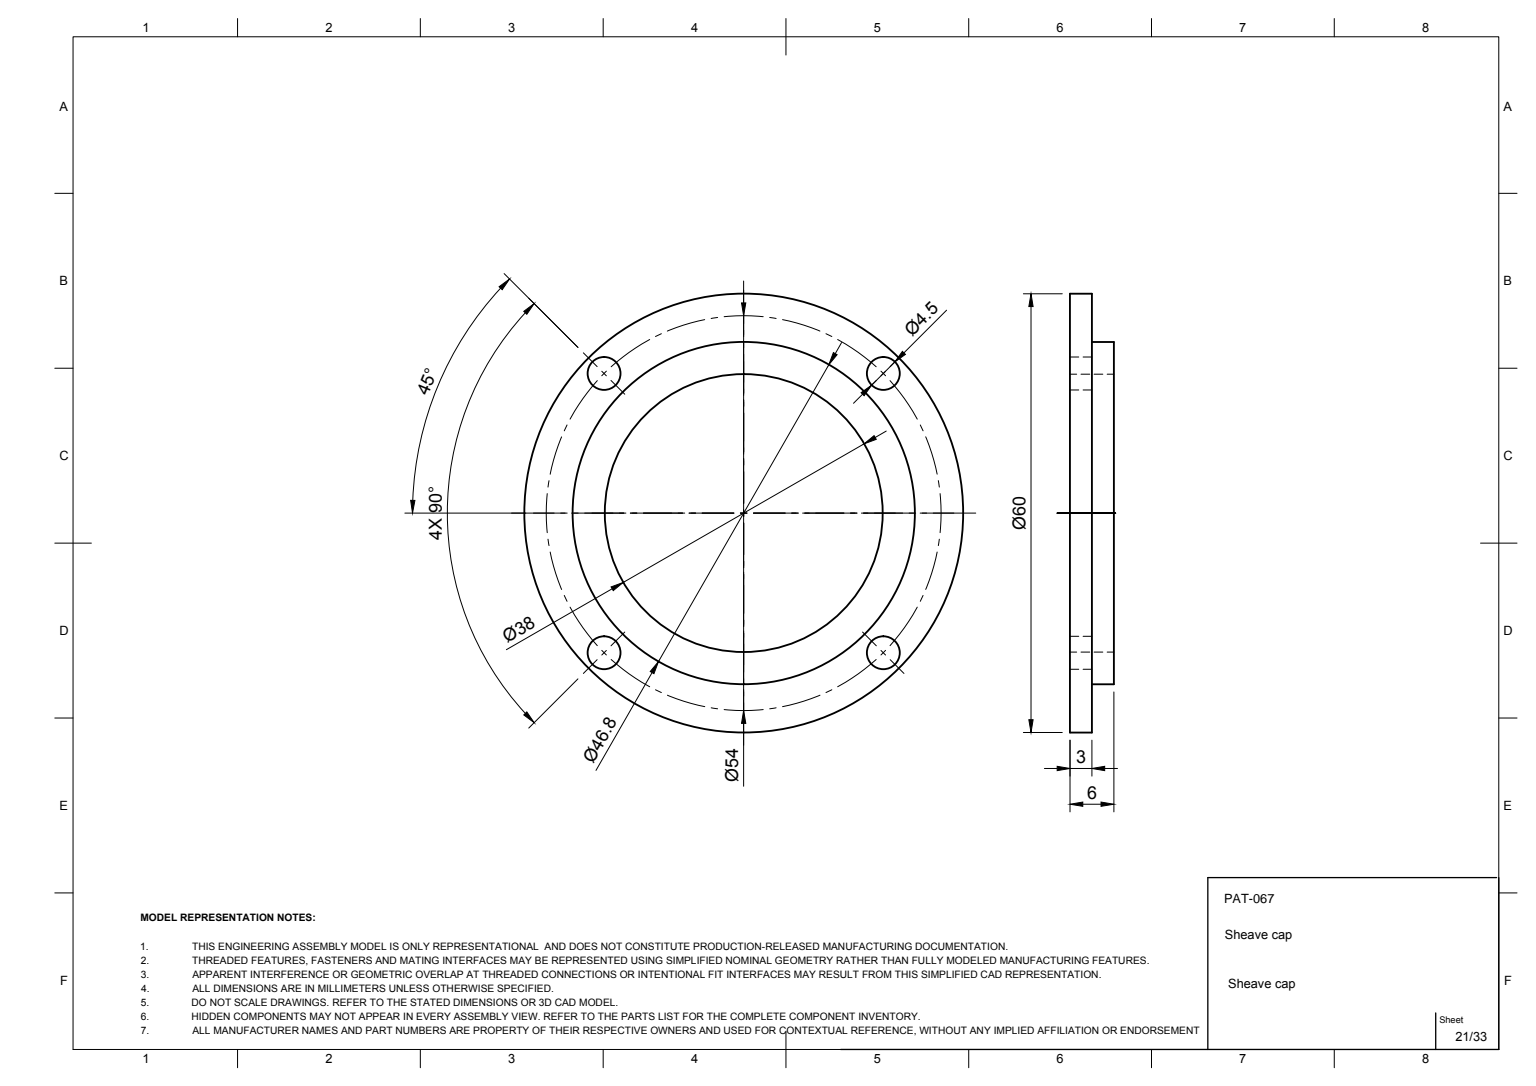
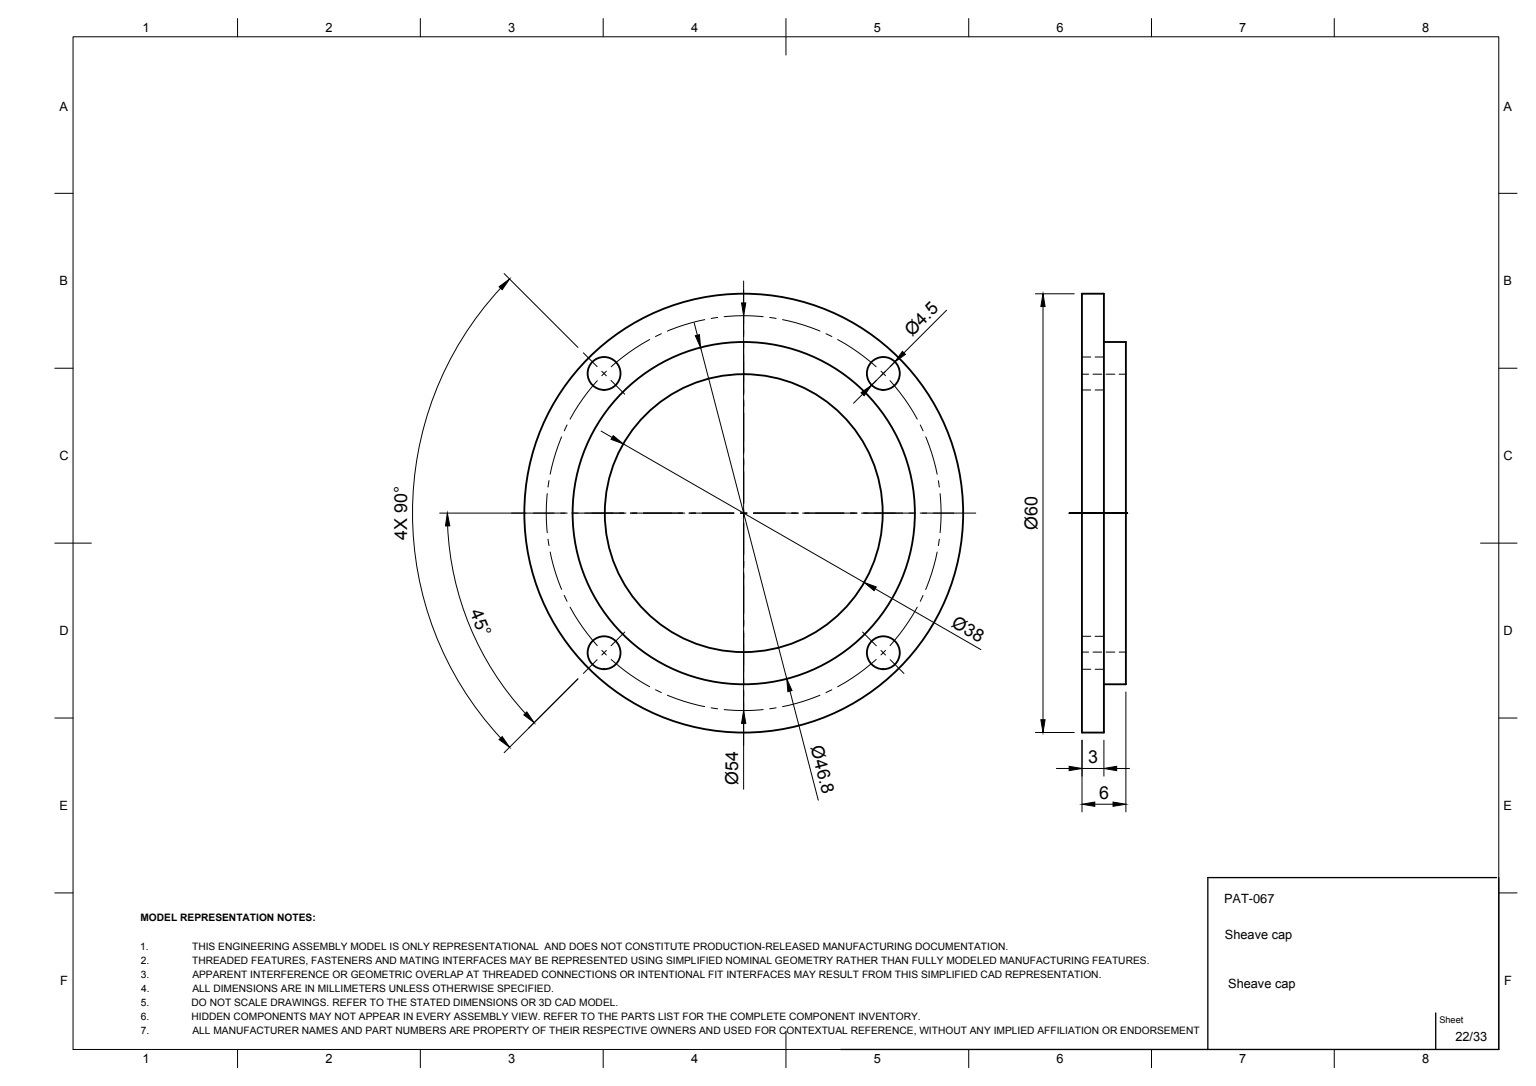
ISO-10303-21;
HEADER;
/* Generated by software containing ST-Developer
 * from STEP Tools, Inc. (www.steptools.com) 
 */

FILE_DESCRIPTION(
/* description */ ('Lifting hook block with sheave'),
/* implementation_level */ '2;1');

FILE_NAME(
/* name */ 'Sheave cap.step',
/* time_stamp */ '2026-10-28T03:23:54-07:00',
/* author */ (''),
/* organization */ (''),
/* preprocessor_version */ 'ST-DEVELOPER v20.2',
/* originating_system */ 'Autodesk Translation Framework v15.17.0.0',
/* authorisation */ '');

FILE_SCHEMA (('AUTOMOTIVE_DESIGN { 1 0 10303 214 3 1 1 }'));
ENDSEC;

DATA;
#10=MECHANICAL_DESIGN_GEOMETRIC_PRESENTATION_REPRESENTATION('',(#369),#9391);
#309=SHAPE_REPRESENTATION_RELATIONSHIP('SRR','None',#9541,#339);
#339=ADVANCED_BREP_SHAPE_REPRESENTATION('',(#405),#9376);
#369=STYLED_ITEM('',(#9773),#405);
#405=MANIFOLD_SOLID_BREP('Body1',#4907);
#612=LINE('',#8395,#900);
#613=LINE('',#8401,#901);
#614=LINE('',#8407,#902);
#615=LINE('',#8413,#903);
#616=LINE('',#8419,#904);
#617=LINE('',#8426,#905);
#618=LINE('',#8432,#906);
#900=VECTOR('',#6869,0.225);
#901=VECTOR('',#6876,0.225);
#902=VECTOR('',#6883,0.225);
#903=VECTOR('',#6890,0.225);
#904=VECTOR('',#6897,2.34);
#905=VECTOR('',#6906,1.9);
#906=VECTOR('',#6913,3.);
#1067=CYLINDRICAL_SURFACE('',#5633,0.225);
#1068=CYLINDRICAL_SURFACE('',#5636,0.225);
#1069=CYLINDRICAL_SURFACE('',#5639,0.225);
#1070=CYLINDRICAL_SURFACE('',#5642,0.225);
#1071=CYLINDRICAL_SURFACE('',#5645,2.34);
#1072=CYLINDRICAL_SURFACE('',#5650,1.9);
#1073=CYLINDRICAL_SURFACE('',#5652,3.);
#1180=FACE_BOUND('',#1757,.T.);
#1181=FACE_BOUND('',#1761,.T.);
#1182=FACE_BOUND('',#1762,.T.);
#1183=FACE_BOUND('',#1763,.T.);
#1184=FACE_BOUND('',#1764,.T.);
#1185=FACE_BOUND('',#1765,.T.);
#1186=FACE_BOUND('',#1767,.T.);
#1187=FACE_BOUND('',#1768,.T.);
#1188=FACE_BOUND('',#1769,.T.);
#1189=FACE_BOUND('',#1770,.T.);
#1190=FACE_BOUND('',#1771,.T.);
#1389=FACE_OUTER_BOUND('',#1751,.T.);
#1390=FACE_OUTER_BOUND('',#1752,.T.);
#1391=FACE_OUTER_BOUND('',#1753,.T.);
#1392=FACE_OUTER_BOUND('',#1754,.T.);
#1393=FACE_OUTER_BOUND('',#1755,.T.);
#1394=FACE_OUTER_BOUND('',#1756,.T.);
#1395=FACE_OUTER_BOUND('',#1758,.T.);
#1396=FACE_OUTER_BOUND('',#1759,.T.);
#1397=FACE_OUTER_BOUND('',#1760,.T.);
#1398=FACE_OUTER_BOUND('',#1766,.T.);
#1751=EDGE_LOOP('',(#3950,#3951,#3952,#3953));
#1752=EDGE_LOOP('',(#3954,#3955,#3956,#3957));
#1753=EDGE_LOOP('',(#3958,#3959,#3960,#3961));
#1754=EDGE_LOOP('',(#3962,#3963,#3964,#3965));
#1755=EDGE_LOOP('',(#3966,#3967,#3968,#3969));
#1756=EDGE_LOOP('',(#3970));
#1757=EDGE_LOOP('',(#3971));
#1758=EDGE_LOOP('',(#3972,#3973,#3974,#3975));
#1759=EDGE_LOOP('',(#3976,#3977,#3978,#3979));
#1760=EDGE_LOOP('',(#3980));
#1761=EDGE_LOOP('',(#3981));
#1762=EDGE_LOOP('',(#3982));
#1763=EDGE_LOOP('',(#3983));
#1764=EDGE_LOOP('',(#3984));
#1765=EDGE_LOOP('',(#3985));
#1766=EDGE_LOOP('',(#3986));
#1767=EDGE_LOOP('',(#3987));
#1768=EDGE_LOOP('',(#3988));
#1769=EDGE_LOOP('',(#3989));
#1770=EDGE_LOOP('',(#3990));
#1771=EDGE_LOOP('',(#3991));
#2075=CIRCLE('',#5634,0.225);
#2076=CIRCLE('',#5635,0.225);
#2077=CIRCLE('',#5637,0.225);
#2078=CIRCLE('',#5638,0.225);
#2079=CIRCLE('',#5640,0.225);
#2080=CIRCLE('',#5641,0.225);
#2081=CIRCLE('',#5643,0.225);
#2082=CIRCLE('',#5644,0.225);
#2083=CIRCLE('',#5646,2.34);
#2084=CIRCLE('',#5647,2.34);
#2085=CIRCLE('',#5649,1.9);
#2086=CIRCLE('',#5651,1.9);
#2087=CIRCLE('',#5653,3.);
#2088=CIRCLE('',#5654,3.);
#2444=VERTEX_POINT('',#8392);
#2445=VERTEX_POINT('',#8394);
#2446=VERTEX_POINT('',#8398);
#2447=VERTEX_POINT('',#8400);
#2448=VERTEX_POINT('',#8404);
#2449=VERTEX_POINT('',#8406);
#2450=VERTEX_POINT('',#8410);
#2451=VERTEX_POINT('',#8412);
#2452=VERTEX_POINT('',#8416);
#2453=VERTEX_POINT('',#8418);
#2454=VERTEX_POINT('',#8422);
#2455=VERTEX_POINT('',#8425);
#2456=VERTEX_POINT('',#8429);
#2457=VERTEX_POINT('',#8431);
#2979=EDGE_CURVE('',#2444,#2444,#2075,.T.);
#2980=EDGE_CURVE('',#2444,#2445,#612,.T.);
#2981=EDGE_CURVE('',#2445,#2445,#2076,.T.);
#2982=EDGE_CURVE('',#2446,#2446,#2077,.T.);
#2983=EDGE_CURVE('',#2446,#2447,#613,.T.);
#2984=EDGE_CURVE('',#2447,#2447,#2078,.T.);
#2985=EDGE_CURVE('',#2448,#2448,#2079,.T.);
#2986=EDGE_CURVE('',#2448,#2449,#614,.T.);
#2987=EDGE_CURVE('',#2449,#2449,#2080,.T.);
#2988=EDGE_CURVE('',#2450,#2450,#2081,.T.);
#2989=EDGE_CURVE('',#2450,#2451,#615,.T.);
#2990=EDGE_CURVE('',#2451,#2451,#2082,.T.);
#2991=EDGE_CURVE('',#2452,#2452,#2083,.T.);
#2992=EDGE_CURVE('',#2452,#2453,#616,.T.);
#2993=EDGE_CURVE('',#2453,#2453,#2084,.T.);
#2994=EDGE_CURVE('',#2454,#2454,#2085,.T.);
#2995=EDGE_CURVE('',#2454,#2455,#617,.T.);
#2996=EDGE_CURVE('',#2455,#2455,#2086,.T.);
#2997=EDGE_CURVE('',#2456,#2456,#2087,.T.);
#2998=EDGE_CURVE('',#2456,#2457,#618,.T.);
#2999=EDGE_CURVE('',#2457,#2457,#2088,.T.);
#3950=ORIENTED_EDGE('',*,*,#2979,.F.);
#3951=ORIENTED_EDGE('',*,*,#2980,.T.);
#3952=ORIENTED_EDGE('',*,*,#2981,.F.);
#3953=ORIENTED_EDGE('',*,*,#2980,.F.);
#3954=ORIENTED_EDGE('',*,*,#2982,.F.);
#3955=ORIENTED_EDGE('',*,*,#2983,.T.);
#3956=ORIENTED_EDGE('',*,*,#2984,.F.);
#3957=ORIENTED_EDGE('',*,*,#2983,.F.);
#3958=ORIENTED_EDGE('',*,*,#2985,.F.);
#3959=ORIENTED_EDGE('',*,*,#2986,.T.);
#3960=ORIENTED_EDGE('',*,*,#2987,.F.);
#3961=ORIENTED_EDGE('',*,*,#2986,.F.);
#3962=ORIENTED_EDGE('',*,*,#2988,.F.);
#3963=ORIENTED_EDGE('',*,*,#2989,.T.);
#3964=ORIENTED_EDGE('',*,*,#2990,.F.);
#3965=ORIENTED_EDGE('',*,*,#2989,.F.);
#3966=ORIENTED_EDGE('',*,*,#2991,.F.);
#3967=ORIENTED_EDGE('',*,*,#2992,.T.);
#3968=ORIENTED_EDGE('',*,*,#2993,.F.);
#3969=ORIENTED_EDGE('',*,*,#2992,.F.);
#3970=ORIENTED_EDGE('',*,*,#2991,.T.);
#3971=ORIENTED_EDGE('',*,*,#2994,.T.);
#3972=ORIENTED_EDGE('',*,*,#2994,.F.);
#3973=ORIENTED_EDGE('',*,*,#2995,.T.);
#3974=ORIENTED_EDGE('',*,*,#2996,.T.);
#3975=ORIENTED_EDGE('',*,*,#2995,.F.);
#3976=ORIENTED_EDGE('',*,*,#2997,.F.);
#3977=ORIENTED_EDGE('',*,*,#2998,.T.);
#3978=ORIENTED_EDGE('',*,*,#2999,.T.);
#3979=ORIENTED_EDGE('',*,*,#2998,.F.);
#3980=ORIENTED_EDGE('',*,*,#2997,.T.);
#3981=ORIENTED_EDGE('',*,*,#2993,.T.);
#3982=ORIENTED_EDGE('',*,*,#2990,.T.);
#3983=ORIENTED_EDGE('',*,*,#2987,.T.);
#3984=ORIENTED_EDGE('',*,*,#2984,.T.);
#3985=ORIENTED_EDGE('',*,*,#2981,.T.);
#3986=ORIENTED_EDGE('',*,*,#2999,.F.);
#3987=ORIENTED_EDGE('',*,*,#2996,.F.);
#3988=ORIENTED_EDGE('',*,*,#2988,.T.);
#3989=ORIENTED_EDGE('',*,*,#2985,.T.);
#3990=ORIENTED_EDGE('',*,*,#2982,.T.);
#3991=ORIENTED_EDGE('',*,*,#2979,.T.);
#4541=PLANE('',#5648);
#4542=PLANE('',#5655);
#4543=PLANE('',#5656);
#4765=ADVANCED_FACE('',(#1389),#1067,.F.);
#4766=ADVANCED_FACE('',(#1390),#1068,.F.);
#4767=ADVANCED_FACE('',(#1391),#1069,.F.);
#4768=ADVANCED_FACE('',(#1392),#1070,.F.);
#4769=ADVANCED_FACE('',(#1393),#1071,.T.);
#4770=ADVANCED_FACE('',(#1394,#1180),#4541,.T.);
#4771=ADVANCED_FACE('',(#1395),#1072,.F.);
#4772=ADVANCED_FACE('',(#1396),#1073,.T.);
#4773=ADVANCED_FACE('',(#1397,#1181,#1182,#1183,#1184,#1185),#4542,.T.);
#4774=ADVANCED_FACE('',(#1398,#1186,#1187,#1188,#1189,#1190),#4543,.F.);
#4907=CLOSED_SHELL('',(#4765,#4766,#4767,#4768,#4769,#4770,#4771,#4772,
#4773,#4774));
#5632=AXIS2_PLACEMENT_3D('',#8390,#6863,#6864);
#5633=AXIS2_PLACEMENT_3D('',#8391,#6865,#6866);
#5634=AXIS2_PLACEMENT_3D('',#8393,#6867,#6868);
#5635=AXIS2_PLACEMENT_3D('',#8396,#6870,#6871);
#5636=AXIS2_PLACEMENT_3D('',#8397,#6872,#6873);
#5637=AXIS2_PLACEMENT_3D('',#8399,#6874,#6875);
#5638=AXIS2_PLACEMENT_3D('',#8402,#6877,#6878);
#5639=AXIS2_PLACEMENT_3D('',#8403,#6879,#6880);
#5640=AXIS2_PLACEMENT_3D('',#8405,#6881,#6882);
#5641=AXIS2_PLACEMENT_3D('',#8408,#6884,#6885);
#5642=AXIS2_PLACEMENT_3D('',#8409,#6886,#6887);
#5643=AXIS2_PLACEMENT_3D('',#8411,#6888,#6889);
#5644=AXIS2_PLACEMENT_3D('',#8414,#6891,#6892);
#5645=AXIS2_PLACEMENT_3D('',#8415,#6893,#6894);
#5646=AXIS2_PLACEMENT_3D('',#8417,#6895,#6896);
#5647=AXIS2_PLACEMENT_3D('',#8420,#6898,#6899);
#5648=AXIS2_PLACEMENT_3D('',#8421,#6900,#6901);
#5649=AXIS2_PLACEMENT_3D('',#8423,#6902,#6903);
#5650=AXIS2_PLACEMENT_3D('',#8424,#6904,#6905);
#5651=AXIS2_PLACEMENT_3D('',#8427,#6907,#6908);
#5652=AXIS2_PLACEMENT_3D('',#8428,#6909,#6910);
#5653=AXIS2_PLACEMENT_3D('',#8430,#6911,#6912);
#5654=AXIS2_PLACEMENT_3D('',#8433,#6914,#6915);
#5655=AXIS2_PLACEMENT_3D('',#8434,#6916,#6917);
#5656=AXIS2_PLACEMENT_3D('',#8435,#6918,#6919);
#6863=DIRECTION('axis',(0.,0.,1.));
#6864=DIRECTION('refdir',(1.,0.,0.));
#6865=DIRECTION('center_axis',(0.,1.,0.));
#6866=DIRECTION('ref_axis',(1.,0.,0.));
#6867=DIRECTION('center_axis',(0.,1.,0.));
#6868=DIRECTION('ref_axis',(1.,0.,0.));
#6869=DIRECTION('',(0.,1.,0.));
#6870=DIRECTION('center_axis',(0.,-1.,0.));
#6871=DIRECTION('ref_axis',(1.,0.,0.));
#6872=DIRECTION('center_axis',(0.,1.,0.));
#6873=DIRECTION('ref_axis',(1.,0.,0.));
#6874=DIRECTION('center_axis',(0.,1.,0.));
#6875=DIRECTION('ref_axis',(1.,0.,0.));
#6876=DIRECTION('',(0.,1.,0.));
#6877=DIRECTION('center_axis',(0.,-1.,0.));
#6878=DIRECTION('ref_axis',(1.,0.,0.));
#6879=DIRECTION('center_axis',(0.,1.,0.));
#6880=DIRECTION('ref_axis',(1.,0.,0.));
#6881=DIRECTION('center_axis',(0.,1.,0.));
#6882=DIRECTION('ref_axis',(1.,0.,0.));
#6883=DIRECTION('',(0.,1.,0.));
#6884=DIRECTION('center_axis',(0.,-1.,0.));
#6885=DIRECTION('ref_axis',(1.,0.,0.));
#6886=DIRECTION('center_axis',(0.,1.,0.));
#6887=DIRECTION('ref_axis',(1.,0.,0.));
#6888=DIRECTION('center_axis',(0.,1.,0.));
#6889=DIRECTION('ref_axis',(1.,0.,0.));
#6890=DIRECTION('',(0.,1.,0.));
#6891=DIRECTION('center_axis',(0.,-1.,0.));
#6892=DIRECTION('ref_axis',(1.,0.,0.));
#6893=DIRECTION('center_axis',(0.,1.,0.));
#6894=DIRECTION('ref_axis',(1.,0.,0.));
#6895=DIRECTION('center_axis',(0.,1.,0.));
#6896=DIRECTION('ref_axis',(1.,0.,0.));
#6897=DIRECTION('',(0.,-1.,0.));
#6898=DIRECTION('center_axis',(0.,-1.,0.));
#6899=DIRECTION('ref_axis',(1.,0.,0.));
#6900=DIRECTION('center_axis',(0.,1.,0.));
#6901=DIRECTION('ref_axis',(1.,0.,0.));
#6902=DIRECTION('center_axis',(0.,-1.,0.));
#6903=DIRECTION('ref_axis',(1.,0.,0.));
#6904=DIRECTION('center_axis',(0.,1.,0.));
#6905=DIRECTION('ref_axis',(1.,0.,0.));
#6906=DIRECTION('',(0.,-1.,0.));
#6907=DIRECTION('center_axis',(0.,-1.,0.));
#6908=DIRECTION('ref_axis',(1.,0.,0.));
#6909=DIRECTION('center_axis',(0.,1.,0.));
#6910=DIRECTION('ref_axis',(1.,0.,0.));
#6911=DIRECTION('center_axis',(0.,1.,0.));
#6912=DIRECTION('ref_axis',(1.,0.,0.));
#6913=DIRECTION('',(0.,-1.,0.));
#6914=DIRECTION('center_axis',(0.,1.,0.));
#6915=DIRECTION('ref_axis',(1.,0.,0.));
#6916=DIRECTION('center_axis',(0.,1.,0.));
#6917=DIRECTION('ref_axis',(1.,0.,0.));
#6918=DIRECTION('center_axis',(0.,1.,0.));
#6919=DIRECTION('ref_axis',(1.,0.,0.));
#8390=CARTESIAN_POINT('',(0.,0.,0.));
#8391=CARTESIAN_POINT('Origin',(-1.90918830920368,-2.4,10.0908116907963));
#8392=CARTESIAN_POINT('',(-2.13418830920368,-2.3,10.0908116907963));
#8393=CARTESIAN_POINT('Origin',(-1.90918830920368,-2.3,10.0908116907963));
#8394=CARTESIAN_POINT('',(-2.13418830920368,-2.,10.0908116907963));
#8395=CARTESIAN_POINT('',(-2.13418830920368,-2.4,10.0908116907963));
#8396=CARTESIAN_POINT('Origin',(-1.90918830920368,-2.,10.0908116907963));
#8397=CARTESIAN_POINT('Origin',(-1.90918830920368,-2.4,13.9091883092037));
#8398=CARTESIAN_POINT('',(-2.13418830920368,-2.3,13.9091883092037));
#8399=CARTESIAN_POINT('Origin',(-1.90918830920368,-2.3,13.9091883092037));
#8400=CARTESIAN_POINT('',(-2.13418830920368,-2.,13.9091883092037));
#8401=CARTESIAN_POINT('',(-2.13418830920368,-2.4,13.9091883092037));
#8402=CARTESIAN_POINT('Origin',(-1.90918830920368,-2.,13.9091883092037));
#8403=CARTESIAN_POINT('Origin',(1.90918830920368,-2.4,13.9091883092037));
#8404=CARTESIAN_POINT('',(1.68418830920368,-2.3,13.9091883092037));
#8405=CARTESIAN_POINT('Origin',(1.90918830920368,-2.3,13.9091883092037));
#8406=CARTESIAN_POINT('',(1.68418830920368,-2.,13.9091883092037));
#8407=CARTESIAN_POINT('',(1.68418830920368,-2.4,13.9091883092037));
#8408=CARTESIAN_POINT('Origin',(1.90918830920368,-2.,13.9091883092037));
#8409=CARTESIAN_POINT('Origin',(1.90918830920368,-2.4,10.0908116907963));
#8410=CARTESIAN_POINT('',(1.68418830920368,-2.3,10.0908116907963));
#8411=CARTESIAN_POINT('Origin',(1.90918830920368,-2.3,10.0908116907963));
#8412=CARTESIAN_POINT('',(1.68418830920368,-2.,10.0908116907963));
#8413=CARTESIAN_POINT('',(1.68418830920368,-2.4,10.0908116907963));
#8414=CARTESIAN_POINT('Origin',(1.90918830920368,-2.,10.0908116907963));
#8415=CARTESIAN_POINT('Origin',(0.,-2.,12.));
#8416=CARTESIAN_POINT('',(-2.34,-1.7,12.));
#8417=CARTESIAN_POINT('Origin',(0.,-1.7,12.));
#8418=CARTESIAN_POINT('',(-2.34,-2.,12.));
#8419=CARTESIAN_POINT('',(-2.34,-2.,12.));
#8420=CARTESIAN_POINT('Origin',(0.,-2.,12.));
#8421=CARTESIAN_POINT('Origin',(0.,-1.7,12.));
#8422=CARTESIAN_POINT('',(-1.9,-1.7,12.));
#8423=CARTESIAN_POINT('Origin',(0.,-1.7,12.));
#8424=CARTESIAN_POINT('Origin',(0.,-2.3,12.));
#8425=CARTESIAN_POINT('',(-1.9,-2.3,12.));
#8426=CARTESIAN_POINT('',(-1.9,-2.3,12.));
#8427=CARTESIAN_POINT('Origin',(0.,-2.3,12.));
#8428=CARTESIAN_POINT('Origin',(0.,-2.3,12.));
#8429=CARTESIAN_POINT('',(-3.,-2.,12.));
#8430=CARTESIAN_POINT('Origin',(0.,-2.,12.));
#8431=CARTESIAN_POINT('',(-3.,-2.3,12.));
#8432=CARTESIAN_POINT('',(-3.,-2.3,12.));
#8433=CARTESIAN_POINT('Origin',(0.,-2.3,12.));
#8434=CARTESIAN_POINT('Origin',(0.,-2.,12.));
#8435=CARTESIAN_POINT('Origin',(0.,-2.3,12.));
#9339=UNCERTAINTY_MEASURE_WITH_UNIT(LENGTH_MEASURE(0.001),#9392,
'DISTANCE_ACCURACY_VALUE',
'Maximum model space distance between geometric entities at asserted c
onnectivities');
#9354=UNCERTAINTY_MEASURE_WITH_UNIT(LENGTH_MEASURE(0.001),#9392,
'DISTANCE_ACCURACY_VALUE',
'Maximum model space distance between geometric entities at asserted c
onnectivities');
#9376=(
GEOMETRIC_REPRESENTATION_CONTEXT(3)
GLOBAL_UNCERTAINTY_ASSIGNED_CONTEXT((#9339))
GLOBAL_UNIT_ASSIGNED_CONTEXT((#9392,#9394,#9395))
REPRESENTATION_CONTEXT('','3D')
);
#9391=(
GEOMETRIC_REPRESENTATION_CONTEXT(3)
GLOBAL_UNCERTAINTY_ASSIGNED_CONTEXT((#9354))
GLOBAL_UNIT_ASSIGNED_CONTEXT((#9392,#9394,#9395))
REPRESENTATION_CONTEXT('','3D')
);
#9392=(
LENGTH_UNIT()
NAMED_UNIT(*)
SI_UNIT(.CENTI.,.METRE.)
);
#9394=(
NAMED_UNIT(*)
PLANE_ANGLE_UNIT()
SI_UNIT($,.RADIAN.)
);
#9395=(
NAMED_UNIT(*)
SI_UNIT($,.STERADIAN.)
SOLID_ANGLE_UNIT()
);
#9417=SHAPE_DEFINITION_REPRESENTATION(#9478,#9541);
#9478=PRODUCT_DEFINITION_SHAPE('',$,#9578);
#9541=SHAPE_REPRESENTATION('',(#5632),#9376);
#9556=PRODUCT_DEFINITION_CONTEXT('part definition',#9666,'design');
#9578=PRODUCT_DEFINITION('Sheave cap','Sheave cap',#9614,#9556);
#9614=PRODUCT_DEFINITION_FORMATION('',$,#9689);
#9666=APPLICATION_CONTEXT(
'Core Data for Automotive Mechanical Design Process');
#9667=PRODUCT_CONTEXT('part definition',#9666,'mechanical');
#9689=PRODUCT('Sheave cap','Sheave cap','Sheave cap',(#9667));
#9767=COLOUR_RGB('Off White',0.89,0.88,0.83);
#9768=FILL_AREA_STYLE_COLOUR('',#9767);
#9769=FILL_AREA_STYLE('',(#9768));
#9770=SURFACE_STYLE_FILL_AREA(#9769);
#9771=SURFACE_SIDE_STYLE('',(#9770));
#9772=SURFACE_STYLE_USAGE(.BOTH.,#9771);
#9773=PRESENTATION_STYLE_ASSIGNMENT((#9772));
ENDSEC;
END-ISO-10303-21;
